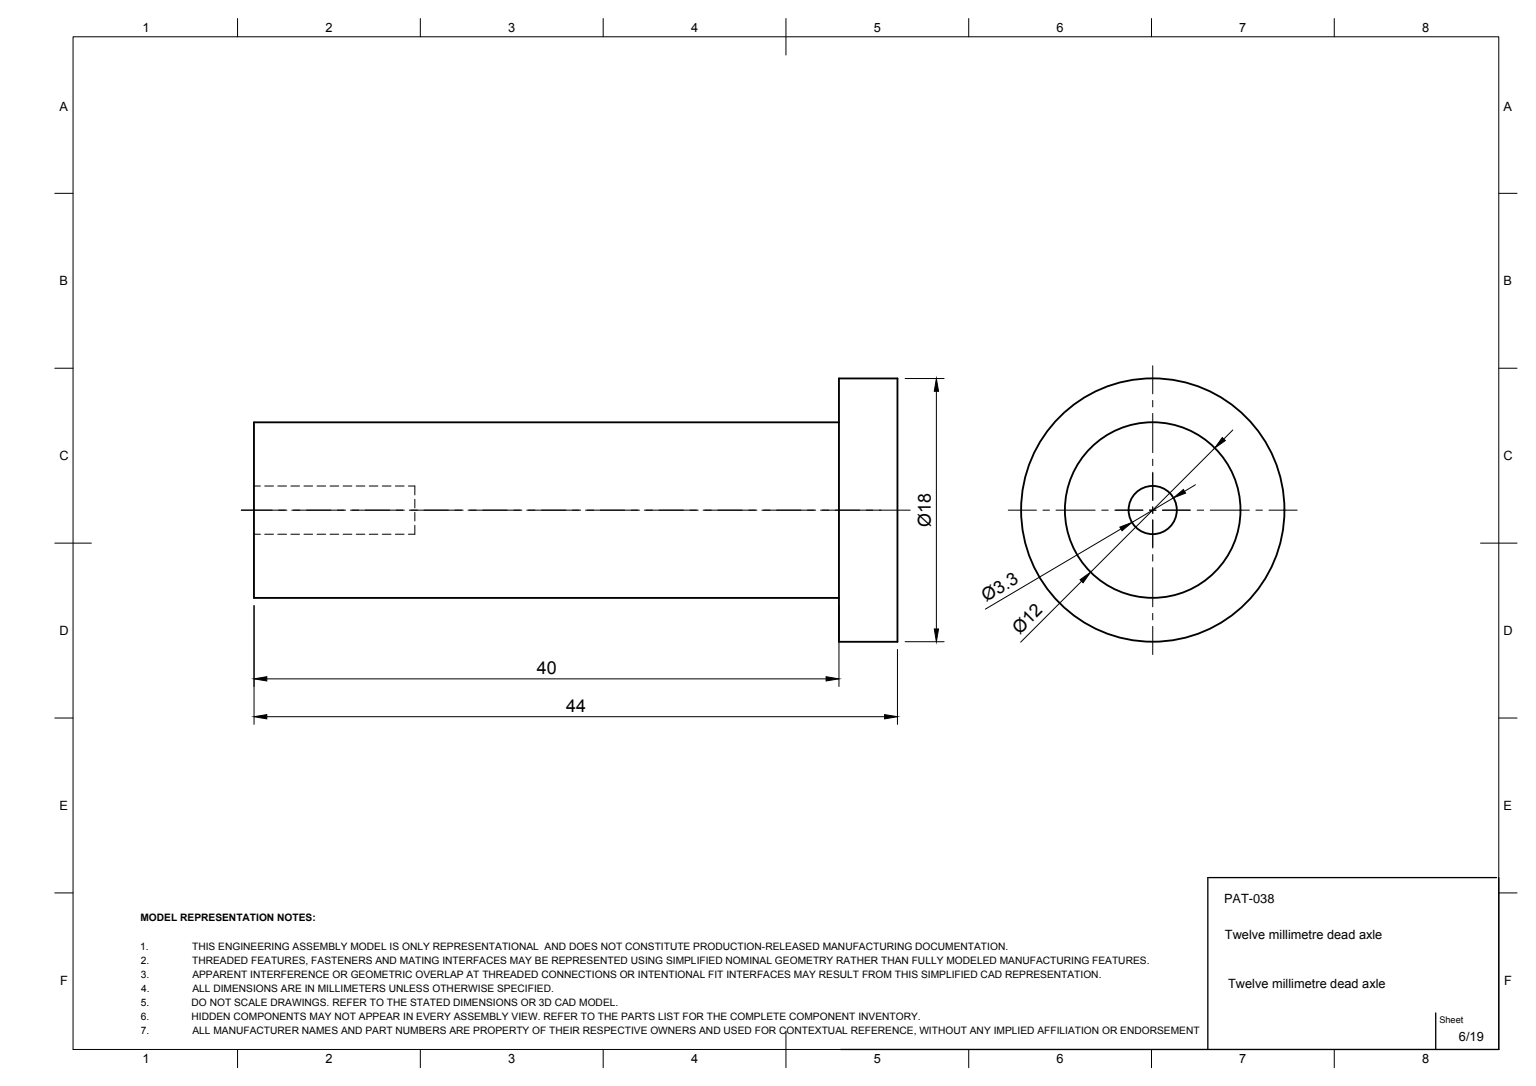
ISO-10303-21;
HEADER;
/* Generated by software containing ST-Developer
 * from STEP Tools, Inc. (www.steptools.com) 
 */

FILE_DESCRIPTION(
/* description */ ('Fork-mounted skate wheel'),
/* implementation_level */ '2;1');

FILE_NAME(
/* name */ 'Twelve millimetre dead axle.step',
/* time_stamp */ '2026-10-29T16:11:26-07:00',
/* author */ (''),
/* organization */ (''),
/* preprocessor_version */ 'ST-DEVELOPER v20.2',
/* originating_system */ 'Autodesk Translation Framework v15.17.0.0',
/* authorisation */ '');

FILE_SCHEMA (('AUTOMOTIVE_DESIGN { 1 0 10303 214 3 1 1 }'));
ENDSEC;

DATA;
#10=MECHANICAL_DESIGN_GEOMETRIC_PRESENTATION_REPRESENTATION('',(#147),#3688);
#123=SHAPE_REPRESENTATION_RELATIONSHIP('SRR','None',#3746,#135);
#135=ADVANCED_BREP_SHAPE_REPRESENTATION('',(#166),#3675);
#147=STYLED_ITEM('',(#3896),#166);
#166=MANIFOLD_SOLID_BREP('Body1',#1808);
#197=FACE_BOUND('',#428,.T.);
#198=FACE_BOUND('',#433,.T.);
#235=PLANE('',#2001);
#236=PLANE('',#2002);
#237=PLANE('',#2007);
#238=PLANE('',#2010);
#298=FACE_OUTER_BOUND('',#425,.T.);
#299=FACE_OUTER_BOUND('',#426,.T.);
#300=FACE_OUTER_BOUND('',#427,.T.);
#301=FACE_OUTER_BOUND('',#429,.T.);
#302=FACE_OUTER_BOUND('',#430,.T.);
#303=FACE_OUTER_BOUND('',#431,.T.);
#304=FACE_OUTER_BOUND('',#432,.T.);
#425=EDGE_LOOP('',(#1325,#1326,#1327,#1328));
#426=EDGE_LOOP('',(#1329));
#427=EDGE_LOOP('',(#1330));
#428=EDGE_LOOP('',(#1331));
#429=EDGE_LOOP('',(#1332,#1333,#1334,#1335));
#430=EDGE_LOOP('',(#1336));
#431=EDGE_LOOP('',(#1337,#1338,#1339,#1340));
#432=EDGE_LOOP('',(#1341));
#433=EDGE_LOOP('',(#1342));
#580=LINE('',#2957,#674);
#581=LINE('',#2967,#675);
#582=LINE('',#2973,#676);
#674=VECTOR('',#2343,0.165);
#675=VECTOR('',#2356,0.9);
#676=VECTOR('',#2365,0.6);
#738=CIRCLE('',#1999,0.165);
#739=CIRCLE('',#2000,0.165);
#740=CIRCLE('',#2003,0.9);
#741=CIRCLE('',#2004,0.6);
#742=CIRCLE('',#2006,0.9);
#743=CIRCLE('',#2009,0.6);
#876=VERTEX_POINT('',#2954);
#877=VERTEX_POINT('',#2956);
#878=VERTEX_POINT('',#2961);
#879=VERTEX_POINT('',#2963);
#880=VERTEX_POINT('',#2966);
#881=VERTEX_POINT('',#2971);
#1049=EDGE_CURVE('',#876,#876,#738,.T.);
#1050=EDGE_CURVE('',#876,#877,#580,.T.);
#1051=EDGE_CURVE('',#877,#877,#739,.T.);
#1052=EDGE_CURVE('',#878,#878,#740,.T.);
#1053=EDGE_CURVE('',#879,#879,#741,.T.);
#1054=EDGE_CURVE('',#878,#880,#581,.T.);
#1055=EDGE_CURVE('',#880,#880,#742,.T.);
#1056=EDGE_CURVE('',#881,#881,#743,.T.);
#1057=EDGE_CURVE('',#881,#879,#582,.T.);
#1325=ORIENTED_EDGE('',*,*,#1049,.F.);
#1326=ORIENTED_EDGE('',*,*,#1050,.T.);
#1327=ORIENTED_EDGE('',*,*,#1051,.F.);
#1328=ORIENTED_EDGE('',*,*,#1050,.F.);
#1329=ORIENTED_EDGE('',*,*,#1049,.T.);
#1330=ORIENTED_EDGE('',*,*,#1052,.T.);
#1331=ORIENTED_EDGE('',*,*,#1053,.F.);
#1332=ORIENTED_EDGE('',*,*,#1052,.F.);
#1333=ORIENTED_EDGE('',*,*,#1054,.T.);
#1334=ORIENTED_EDGE('',*,*,#1055,.T.);
#1335=ORIENTED_EDGE('',*,*,#1054,.F.);
#1336=ORIENTED_EDGE('',*,*,#1055,.F.);
#1337=ORIENTED_EDGE('',*,*,#1056,.F.);
#1338=ORIENTED_EDGE('',*,*,#1057,.T.);
#1339=ORIENTED_EDGE('',*,*,#1053,.T.);
#1340=ORIENTED_EDGE('',*,*,#1057,.F.);
#1341=ORIENTED_EDGE('',*,*,#1056,.T.);
#1342=ORIENTED_EDGE('',*,*,#1051,.T.);
#1667=CYLINDRICAL_SURFACE('',#1998,0.165);
#1668=CYLINDRICAL_SURFACE('',#2005,0.9);
#1669=CYLINDRICAL_SURFACE('',#2008,0.6);
#1716=ADVANCED_FACE('',(#298),#1667,.F.);
#1717=ADVANCED_FACE('',(#299),#235,.T.);
#1718=ADVANCED_FACE('',(#300,#197),#236,.T.);
#1719=ADVANCED_FACE('',(#301),#1668,.T.);
#1720=ADVANCED_FACE('',(#302),#237,.F.);
#1721=ADVANCED_FACE('',(#303),#1669,.T.);
#1722=ADVANCED_FACE('',(#304,#198),#238,.T.);
#1808=CLOSED_SHELL('',(#1716,#1717,#1718,#1719,#1720,#1721,#1722));
#1997=AXIS2_PLACEMENT_3D('',#2952,#2337,#2338);
#1998=AXIS2_PLACEMENT_3D('',#2953,#2339,#2340);
#1999=AXIS2_PLACEMENT_3D('',#2955,#2341,#2342);
#2000=AXIS2_PLACEMENT_3D('',#2958,#2344,#2345);
#2001=AXIS2_PLACEMENT_3D('',#2959,#2346,#2347);
#2002=AXIS2_PLACEMENT_3D('',#2960,#2348,#2349);
#2003=AXIS2_PLACEMENT_3D('',#2962,#2350,#2351);
#2004=AXIS2_PLACEMENT_3D('',#2964,#2352,#2353);
#2005=AXIS2_PLACEMENT_3D('',#2965,#2354,#2355);
#2006=AXIS2_PLACEMENT_3D('',#2968,#2357,#2358);
#2007=AXIS2_PLACEMENT_3D('',#2969,#2359,#2360);
#2008=AXIS2_PLACEMENT_3D('',#2970,#2361,#2362);
#2009=AXIS2_PLACEMENT_3D('',#2972,#2363,#2364);
#2010=AXIS2_PLACEMENT_3D('',#2974,#2366,#2367);
#2337=DIRECTION('axis',(0.,0.,1.));
#2338=DIRECTION('refdir',(1.,0.,0.));
#2339=DIRECTION('center_axis',(0.,1.,0.));
#2340=DIRECTION('ref_axis',(1.,0.,0.));
#2341=DIRECTION('center_axis',(0.,1.,0.));
#2342=DIRECTION('ref_axis',(1.,0.,0.));
#2343=DIRECTION('',(0.,1.,0.));
#2344=DIRECTION('center_axis',(0.,-1.,0.));
#2345=DIRECTION('ref_axis',(1.,0.,0.));
#2346=DIRECTION('center_axis',(0.,1.,0.));
#2347=DIRECTION('ref_axis',(1.,0.,0.));
#2348=DIRECTION('center_axis',(0.,1.,0.));
#2349=DIRECTION('ref_axis',(1.,0.,0.));
#2350=DIRECTION('center_axis',(0.,1.,0.));
#2351=DIRECTION('ref_axis',(1.,0.,0.));
#2352=DIRECTION('center_axis',(0.,1.,0.));
#2353=DIRECTION('ref_axis',(1.,0.,0.));
#2354=DIRECTION('center_axis',(0.,1.,0.));
#2355=DIRECTION('ref_axis',(1.,0.,0.));
#2356=DIRECTION('',(0.,-1.,0.));
#2357=DIRECTION('center_axis',(0.,1.,0.));
#2358=DIRECTION('ref_axis',(1.,0.,0.));
#2359=DIRECTION('center_axis',(0.,1.,0.));
#2360=DIRECTION('ref_axis',(1.,0.,0.));
#2361=DIRECTION('center_axis',(0.,1.,0.));
#2362=DIRECTION('ref_axis',(1.,0.,0.));
#2363=DIRECTION('center_axis',(0.,1.,0.));
#2364=DIRECTION('ref_axis',(1.,0.,0.));
#2365=DIRECTION('',(0.,-1.,0.));
#2366=DIRECTION('center_axis',(0.,1.,0.));
#2367=DIRECTION('ref_axis',(1.,0.,0.));
#2952=CARTESIAN_POINT('',(0.,0.,0.));
#2953=CARTESIAN_POINT('Origin',(0.,0.9,3.5));
#2954=CARTESIAN_POINT('',(-0.165,0.9,3.5));
#2955=CARTESIAN_POINT('Origin',(0.,0.9,3.5));
#2956=CARTESIAN_POINT('',(-0.165,2.,3.5));
#2957=CARTESIAN_POINT('',(-0.165,0.9,3.5));
#2958=CARTESIAN_POINT('Origin',(0.,2.,3.5));
#2959=CARTESIAN_POINT('Origin',(0.,0.9,3.5));
#2960=CARTESIAN_POINT('Origin',(0.,-2.,3.5));
#2961=CARTESIAN_POINT('',(-0.9,-2.,3.5));
#2962=CARTESIAN_POINT('Origin',(0.,-2.,3.5));
#2963=CARTESIAN_POINT('',(-0.6,-2.,3.5));
#2964=CARTESIAN_POINT('Origin',(0.,-2.,3.5));
#2965=CARTESIAN_POINT('Origin',(0.,-2.4,3.5));
#2966=CARTESIAN_POINT('',(-0.9,-2.4,3.5));
#2967=CARTESIAN_POINT('',(-0.9,-2.4,3.5));
#2968=CARTESIAN_POINT('Origin',(0.,-2.4,3.5));
#2969=CARTESIAN_POINT('Origin',(0.,-2.4,3.5));
#2970=CARTESIAN_POINT('Origin',(0.,-2.,3.5));
#2971=CARTESIAN_POINT('',(-0.6,2.,3.5));
#2972=CARTESIAN_POINT('Origin',(0.,2.,3.5));
#2973=CARTESIAN_POINT('',(-0.6,-2.,3.5));
#2974=CARTESIAN_POINT('Origin',(0.,2.,3.5));
#3658=UNCERTAINTY_MEASURE_WITH_UNIT(LENGTH_MEASURE(0.001),#3689,
'DISTANCE_ACCURACY_VALUE',
'Maximum model space distance between geometric entities at asserted c
onnectivities');
#3671=UNCERTAINTY_MEASURE_WITH_UNIT(LENGTH_MEASURE(0.001),#3689,
'DISTANCE_ACCURACY_VALUE',
'Maximum model space distance between geometric entities at asserted c
onnectivities');
#3675=(
GEOMETRIC_REPRESENTATION_CONTEXT(3)
GLOBAL_UNCERTAINTY_ASSIGNED_CONTEXT((#3658))
GLOBAL_UNIT_ASSIGNED_CONTEXT((#3689,#3691,#3692))
REPRESENTATION_CONTEXT('','3D')
);
#3688=(
GEOMETRIC_REPRESENTATION_CONTEXT(3)
GLOBAL_UNCERTAINTY_ASSIGNED_CONTEXT((#3671))
GLOBAL_UNIT_ASSIGNED_CONTEXT((#3689,#3691,#3692))
REPRESENTATION_CONTEXT('','3D')
);
#3689=(
LENGTH_UNIT()
NAMED_UNIT(*)
SI_UNIT(.CENTI.,.METRE.)
);
#3691=(
NAMED_UNIT(*)
PLANE_ANGLE_UNIT()
SI_UNIT($,.RADIAN.)
);
#3692=(
NAMED_UNIT(*)
SI_UNIT($,.STERADIAN.)
SOLID_ANGLE_UNIT()
);
#3696=SHAPE_DEFINITION_REPRESENTATION(#3712,#3746);
#3712=PRODUCT_DEFINITION_SHAPE('',$,#3763);
#3746=SHAPE_REPRESENTATION('',(#1997),#3675);
#3759=PRODUCT_DEFINITION_CONTEXT('part definition',#3809,'design');
#3763=PRODUCT_DEFINITION('Twelve millimetre dead axle',
'Twelve millimetre dead axle',#3779,#3759);
#3779=PRODUCT_DEFINITION_FORMATION('',$,#3814);
#3809=APPLICATION_CONTEXT(
'Core Data for Automotive Mechanical Design Process');
#3810=PRODUCT_CONTEXT('part definition',#3809,'mechanical');
#3814=PRODUCT('Twelve millimetre dead axle',
'Twelve millimetre dead axle','Twelve millimetre dead axle',(#3810));
#3890=COLOUR_RGB('Grey',0.48,0.52,0.57);
#3891=FILL_AREA_STYLE_COLOUR('',#3890);
#3892=FILL_AREA_STYLE('',(#3891));
#3893=SURFACE_STYLE_FILL_AREA(#3892);
#3894=SURFACE_SIDE_STYLE('',(#3893));
#3895=SURFACE_STYLE_USAGE(.BOTH.,#3894);
#3896=PRESENTATION_STYLE_ASSIGNMENT((#3895));
ENDSEC;
END-ISO-10303-21;
